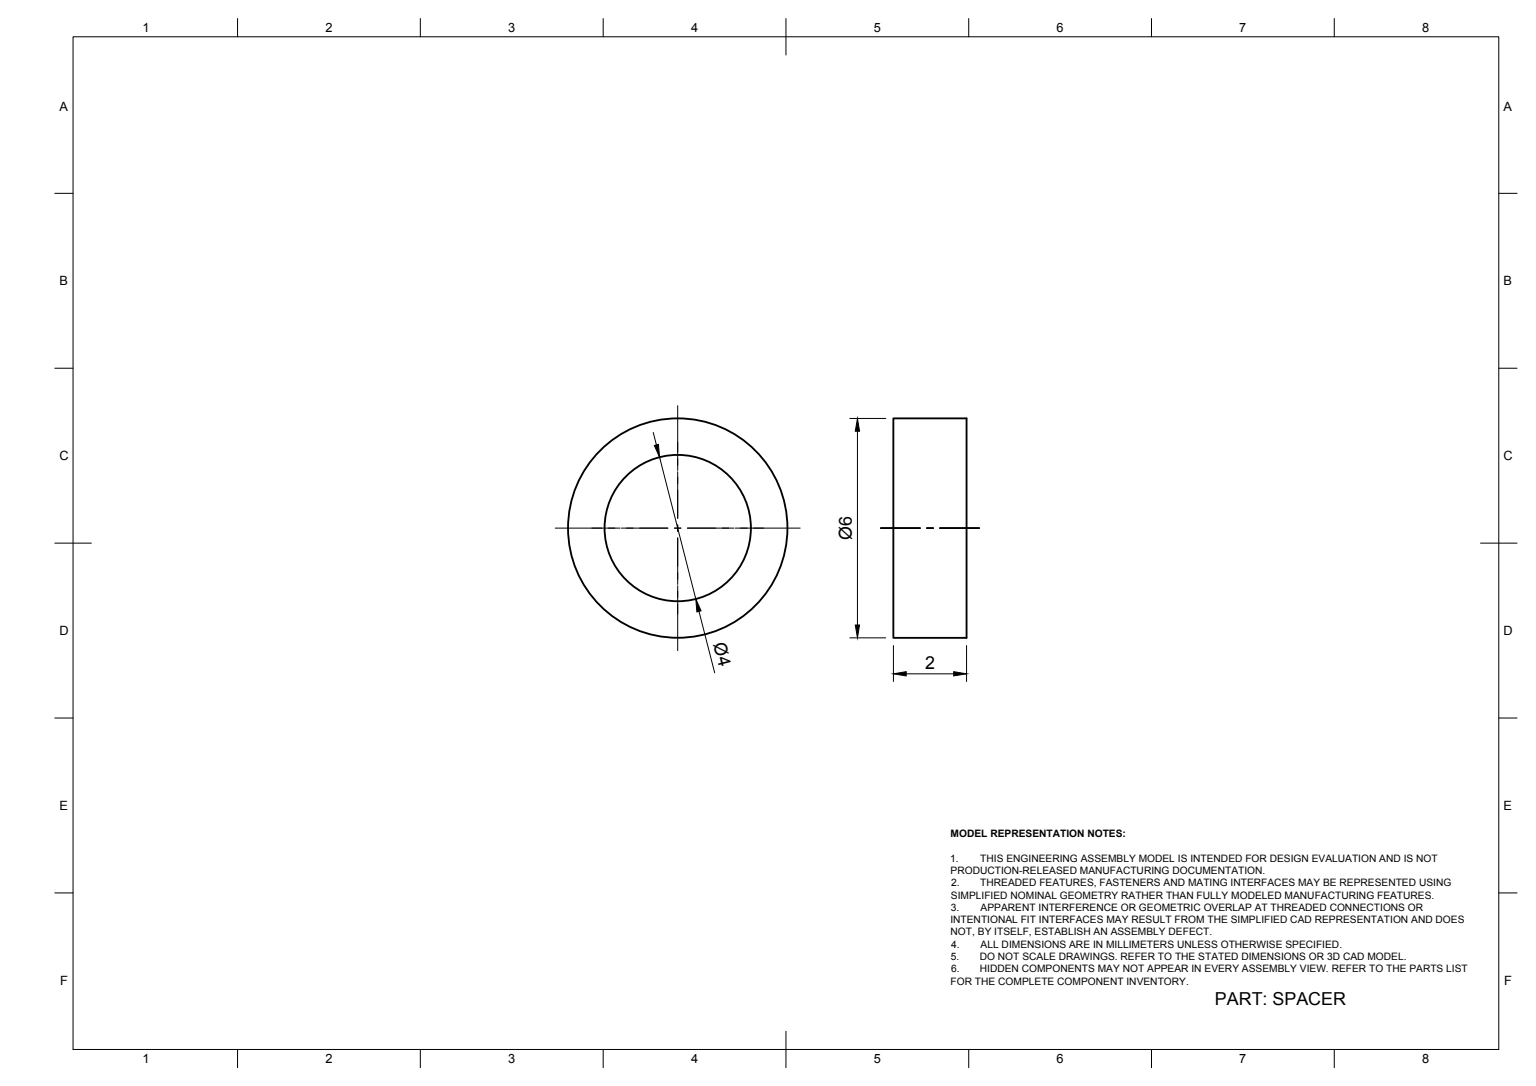
ISO-10303-21;
HEADER;
/* Generated by software containing ST-Developer
 * from STEP Tools, Inc. (www.steptools.com) 
 */

FILE_DESCRIPTION(
/* description */ (''),
/* implementation_level */ '2;1');

FILE_NAME(
/* name */ 'Spacer.step',
/* time_stamp */ '2026-10-04T15:18:51-07:00',
/* author */ (''),
/* organization */ (''),
/* preprocessor_version */ 'ST-DEVELOPER v20.2',
/* originating_system */ 'Autodesk Translation Framework v15.15.0.0',
/* authorisation */ '');

FILE_SCHEMA (('AUTOMOTIVE_DESIGN { 1 0 10303 214 3 1 1 }'));
ENDSEC;

DATA;
#10=MECHANICAL_DESIGN_GEOMETRIC_PRESENTATION_REPRESENTATION('',(#74),#9891);
#55=SHAPE_REPRESENTATION_RELATIONSHIP('SRR','None',#9926,#63);
#63=ADVANCED_BREP_SHAPE_REPRESENTATION('',(#88),#9886);
#74=STYLED_ITEM('',(#9972),#88);
#88=MANIFOLD_SOLID_BREP('Body1',#5622);
#123=FACE_BOUND('',#856,.T.);
#124=FACE_BOUND('',#858,.T.);
#196=PLANE('',#5926);
#197=PLANE('',#5927);
#496=FACE_OUTER_BOUND('',#853,.T.);
#497=FACE_OUTER_BOUND('',#854,.T.);
#498=FACE_OUTER_BOUND('',#855,.T.);
#499=FACE_OUTER_BOUND('',#857,.T.);
#853=EDGE_LOOP('',(#3966,#3967,#3968,#3969));
#854=EDGE_LOOP('',(#3970,#3971,#3972,#3973));
#855=EDGE_LOOP('',(#3974));
#856=EDGE_LOOP('',(#3975));
#857=EDGE_LOOP('',(#3976));
#858=EDGE_LOOP('',(#3977));
#1181=LINE('',#8531,#1645);
#1182=LINE('',#8537,#1646);
#1645=VECTOR('',#6826,1.99999999999999);
#1646=VECTOR('',#6833,2.99999999999999);
#2167=CIRCLE('',#5921,1.99999999999999);
#2168=CIRCLE('',#5922,1.99999999999999);
#2169=CIRCLE('',#5924,2.99999999999999);
#2170=CIRCLE('',#5925,2.99999999999999);
#2463=VERTEX_POINT('',#8528);
#2464=VERTEX_POINT('',#8530);
#2465=VERTEX_POINT('',#8534);
#2466=VERTEX_POINT('',#8536);
#3028=EDGE_CURVE('',#2463,#2463,#2167,.T.);
#3029=EDGE_CURVE('',#2463,#2464,#1181,.T.);
#3030=EDGE_CURVE('',#2464,#2464,#2168,.T.);
#3031=EDGE_CURVE('',#2465,#2465,#2169,.T.);
#3032=EDGE_CURVE('',#2465,#2466,#1182,.T.);
#3033=EDGE_CURVE('',#2466,#2466,#2170,.T.);
#3966=ORIENTED_EDGE('',*,*,#3028,.T.);
#3967=ORIENTED_EDGE('',*,*,#3029,.T.);
#3968=ORIENTED_EDGE('',*,*,#3030,.F.);
#3969=ORIENTED_EDGE('',*,*,#3029,.F.);
#3970=ORIENTED_EDGE('',*,*,#3031,.F.);
#3971=ORIENTED_EDGE('',*,*,#3032,.T.);
#3972=ORIENTED_EDGE('',*,*,#3033,.T.);
#3973=ORIENTED_EDGE('',*,*,#3032,.F.);
#3974=ORIENTED_EDGE('',*,*,#3031,.T.);
#3975=ORIENTED_EDGE('',*,*,#3030,.T.);
#3976=ORIENTED_EDGE('',*,*,#3033,.F.);
#3977=ORIENTED_EDGE('',*,*,#3028,.F.);
#5220=CYLINDRICAL_SURFACE('',#5920,1.99999999999999);
#5221=CYLINDRICAL_SURFACE('',#5923,2.99999999999999);
#5375=ADVANCED_FACE('',(#496),#5220,.F.);
#5376=ADVANCED_FACE('',(#497),#5221,.T.);
#5377=ADVANCED_FACE('',(#498,#123),#196,.T.);
#5378=ADVANCED_FACE('',(#499,#124),#197,.F.);
#5622=CLOSED_SHELL('',(#5375,#5376,#5377,#5378));
#5919=AXIS2_PLACEMENT_3D('',#8526,#6820,#6821);
#5920=AXIS2_PLACEMENT_3D('',#8527,#6822,#6823);
#5921=AXIS2_PLACEMENT_3D('',#8529,#6824,#6825);
#5922=AXIS2_PLACEMENT_3D('',#8532,#6827,#6828);
#5923=AXIS2_PLACEMENT_3D('',#8533,#6829,#6830);
#5924=AXIS2_PLACEMENT_3D('',#8535,#6831,#6832);
#5925=AXIS2_PLACEMENT_3D('',#8538,#6834,#6835);
#5926=AXIS2_PLACEMENT_3D('',#8539,#6836,#6837);
#5927=AXIS2_PLACEMENT_3D('',#8540,#6838,#6839);
#6820=DIRECTION('axis',(0.,0.,1.));
#6821=DIRECTION('refdir',(1.,0.,0.));
#6822=DIRECTION('center_axis',(-1.38777878078145E-16,-1.,0.));
#6823=DIRECTION('ref_axis',(1.,-1.38777878078145E-16,-1.5395124730131E-48));
#6824=DIRECTION('center_axis',(8.32667268468864E-17,1.,2.13821176807379E-50));
#6825=DIRECTION('ref_axis',(1.,-8.32667268468864E-17,-1.5395124730131E-48));
#6826=DIRECTION('',(-1.38777878078145E-16,-1.,0.));
#6827=DIRECTION('center_axis',(8.32667268468864E-17,1.,2.13821176807379E-50));
#6828=DIRECTION('ref_axis',(1.,-8.32667268468864E-17,-1.5395124730131E-48));
#6829=DIRECTION('center_axis',(-1.38777878078145E-16,-1.,0.));
#6830=DIRECTION('ref_axis',(1.,-1.38777878078145E-16,-1.5395124730131E-48));
#6831=DIRECTION('center_axis',(-8.32667268468864E-17,-1.,-2.13821176807379E-50));
#6832=DIRECTION('ref_axis',(1.,-8.32667268468864E-17,-1.5395124730131E-48));
#6833=DIRECTION('',(1.38777878078145E-16,1.,0.));
#6834=DIRECTION('center_axis',(-8.32667268468864E-17,-1.,-2.13821176807379E-50));
#6835=DIRECTION('ref_axis',(1.,-8.32667268468864E-17,-1.5395124730131E-48));
#6836=DIRECTION('center_axis',(-8.32667268468864E-17,-1.,-2.13821176807379E-50));
#6837=DIRECTION('ref_axis',(1.,-8.32667268468864E-17,-1.5395124730131E-48));
#6838=DIRECTION('center_axis',(-8.32667268468864E-17,-1.,-2.13821176807379E-50));
#6839=DIRECTION('ref_axis',(1.,-8.32667268468864E-17,-1.5395124730131E-48));
#8526=CARTESIAN_POINT('',(0.,0.,0.));
#8527=CARTESIAN_POINT('Origin',(3.64981768126446E-16,-4.00000000000001,
86.8));
#8528=CARTESIAN_POINT('',(-1.99999999999999,-4.00000000000001,86.8));
#8529=CARTESIAN_POINT('Origin',(3.64981768126446E-16,-4.00000000000001,
86.8));
#8530=CARTESIAN_POINT('',(-1.99999999999999,-6.00000000000001,86.8));
#8531=CARTESIAN_POINT('',(-1.99999999999999,-4.00000000000001,86.8));
#8532=CARTESIAN_POINT('Origin',(8.74260119701567E-17,-6.00000000000001,
86.8));
#8533=CARTESIAN_POINT('Origin',(3.64981768126446E-16,-4.00000000000001,
86.8));
#8534=CARTESIAN_POINT('',(-2.99999999999999,-6.00000000000001,86.8));
#8535=CARTESIAN_POINT('Origin',(8.74260119701567E-17,-6.00000000000001,
86.8));
#8536=CARTESIAN_POINT('',(-2.99999999999999,-4.00000000000001,86.8));
#8537=CARTESIAN_POINT('',(-2.99999999999999,-4.00000000000001,86.8));
#8538=CARTESIAN_POINT('Origin',(3.64981768126446E-16,-4.00000000000001,
86.8));
#8539=CARTESIAN_POINT('Origin',(-5.55111416207579E-17,-6.00000000000001,
86.8));
#8540=CARTESIAN_POINT('Origin',(2.22044614535531E-16,-4.00000000000001,
86.8));
#9876=UNCERTAINTY_MEASURE_WITH_UNIT(LENGTH_MEASURE(0.01),#9892,
'DISTANCE_ACCURACY_VALUE',
'Maximum model space distance between geometric entities at asserted c
onnectivities');
#9881=UNCERTAINTY_MEASURE_WITH_UNIT(LENGTH_MEASURE(0.01),#9892,
'DISTANCE_ACCURACY_VALUE',
'Maximum model space distance between geometric entities at asserted c
onnectivities');
#9886=(
GEOMETRIC_REPRESENTATION_CONTEXT(3)
GLOBAL_UNCERTAINTY_ASSIGNED_CONTEXT((#9876))
GLOBAL_UNIT_ASSIGNED_CONTEXT((#9892,#9894,#9895))
REPRESENTATION_CONTEXT('','3D')
);
#9891=(
GEOMETRIC_REPRESENTATION_CONTEXT(3)
GLOBAL_UNCERTAINTY_ASSIGNED_CONTEXT((#9881))
GLOBAL_UNIT_ASSIGNED_CONTEXT((#9892,#9894,#9895))
REPRESENTATION_CONTEXT('','3D')
);
#9892=(
LENGTH_UNIT()
NAMED_UNIT(*)
SI_UNIT(.MILLI.,.METRE.)
);
#9894=(
NAMED_UNIT(*)
PLANE_ANGLE_UNIT()
SI_UNIT($,.RADIAN.)
);
#9895=(
NAMED_UNIT(*)
SI_UNIT($,.STERADIAN.)
SOLID_ANGLE_UNIT()
);
#9900=SHAPE_DEFINITION_REPRESENTATION(#9909,#9926);
#9909=PRODUCT_DEFINITION_SHAPE('',$,#9936);
#9926=SHAPE_REPRESENTATION('',(#5919),#9886);
#9931=PRODUCT_DEFINITION_CONTEXT('part definition',#9960,'design');
#9936=PRODUCT_DEFINITION('spacer','Spacer',#9945,#9931);
#9945=PRODUCT_DEFINITION_FORMATION('',$,#9966);
#9960=APPLICATION_CONTEXT(
'Core Data for Automotive Mechanical Design Process');
#9961=PRODUCT_CONTEXT('part definition',#9960,'mechanical');
#9966=PRODUCT('spacer','Spacer',$,(#9961));
#9972=PRESENTATION_STYLE_ASSIGNMENT((#9977));
#9977=SURFACE_STYLE_USAGE(.BOTH.,#9982);
#9982=SURFACE_SIDE_STYLE('',(#9987));
#9987=SURFACE_STYLE_FILL_AREA(#9992);
#9992=FILL_AREA_STYLE('Opaque(160,160,160)',(#9997));
#9997=FILL_AREA_STYLE_COLOUR('Opaque(160,160,160)',#10002);
#10002=COLOUR_RGB('Opaque(160,160,160)', 0.09019608, 0.27058824, 0.51372549);
ENDSEC;
END-ISO-10303-21;
